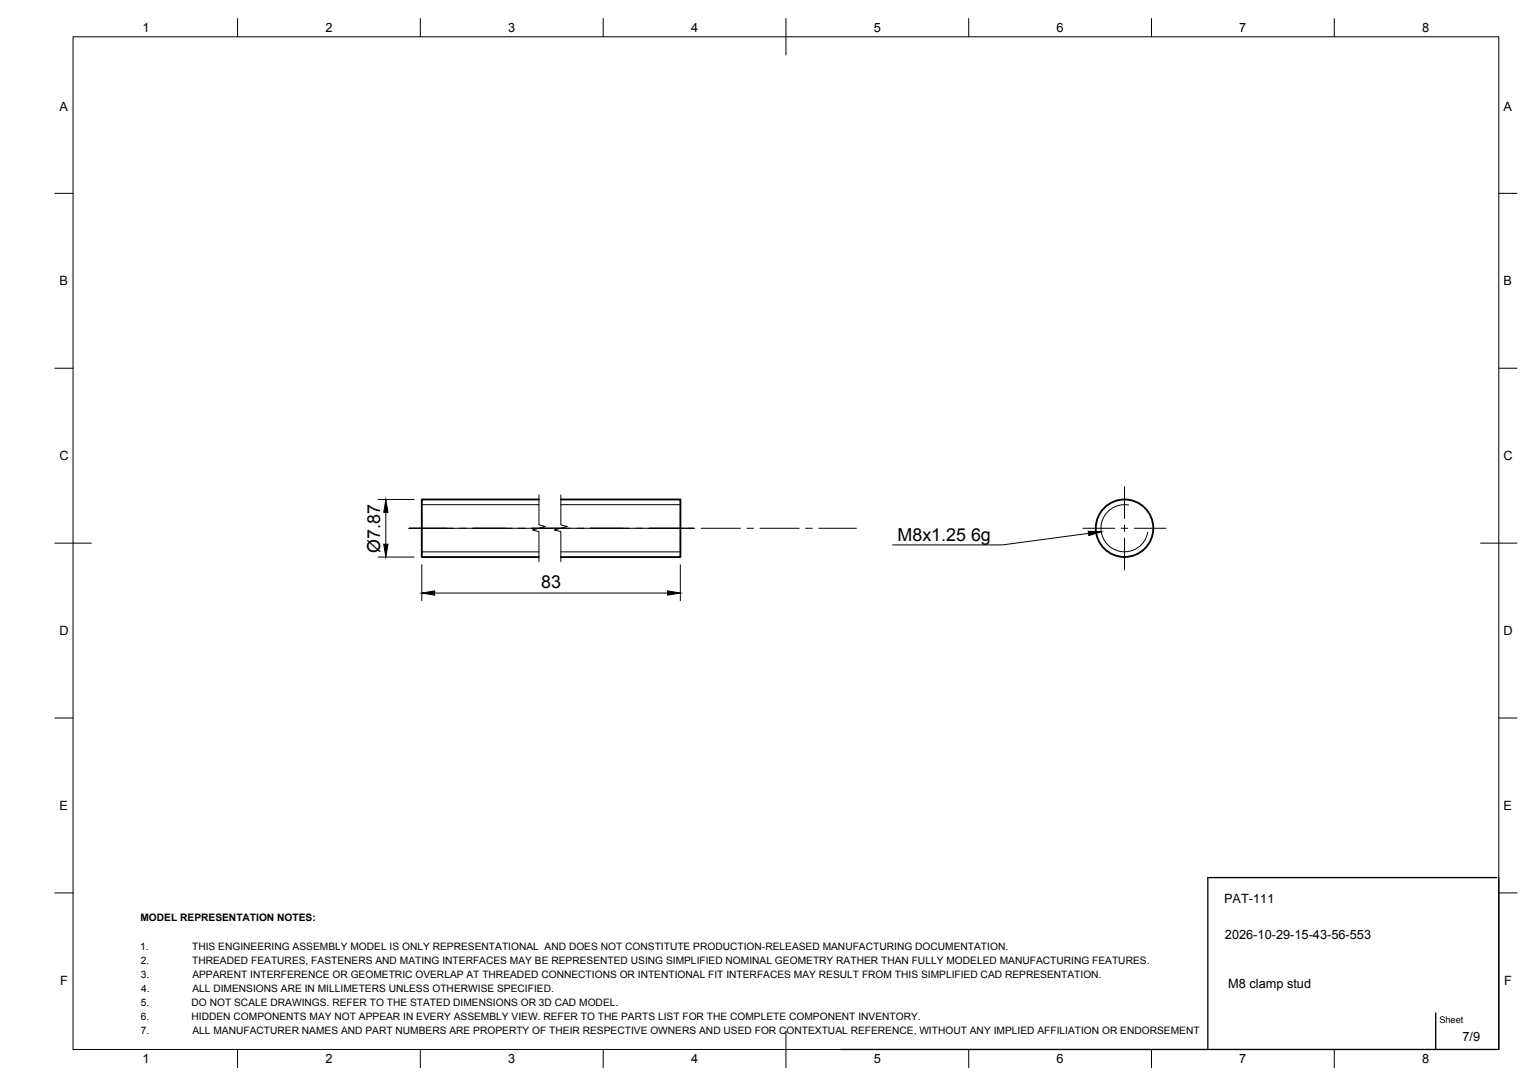
ISO-10303-21;
HEADER;
/* Generated by software containing ST-Developer
 * from STEP Tools, Inc. (www.steptools.com) 
 */

FILE_DESCRIPTION(
/* description */ ('Grid plate located blocks and clamp'),
/* implementation_level */ '2;1');

FILE_NAME(
/* name */ 'M8 clamp stud.step',
/* time_stamp */ '2026-10-29T15:43:47-07:00',
/* author */ (''),
/* organization */ (''),
/* preprocessor_version */ 'ST-DEVELOPER v20.2',
/* originating_system */ 'Autodesk Translation Framework v15.17.0.0',
/* authorisation */ '');

FILE_SCHEMA (('AUTOMOTIVE_DESIGN { 1 0 10303 214 3 1 1 }'));
ENDSEC;

DATA;
#10=MECHANICAL_DESIGN_GEOMETRIC_PRESENTATION_REPRESENTATION('',(#176),#5702);
#150=SHAPE_REPRESENTATION_RELATIONSHIP('SRR','None',#5768,#162);
#162=ADVANCED_BREP_SHAPE_REPRESENTATION('',(#188),#5698);
#176=STYLED_ITEM('',(#5904),#188);
#188=MANIFOLD_SOLID_BREP('Body1',#3273);
#361=CIRCLE('',#3659,0.3933);
#362=CIRCLE('',#3660,0.3933);
#440=CYLINDRICAL_SURFACE('',#3658,0.3933);
#600=FACE_OUTER_BOUND('',#852,.T.);
#601=FACE_OUTER_BOUND('',#853,.T.);
#602=FACE_OUTER_BOUND('',#854,.T.);
#852=EDGE_LOOP('',(#2782,#2783,#2784,#2785));
#853=EDGE_LOOP('',(#2786));
#854=EDGE_LOOP('',(#2787));
#1129=LINE('',#5435,#1402);
#1402=VECTOR('',#4493,0.4);
#1656=VERTEX_POINT('',#5432);
#1657=VERTEX_POINT('',#5434);
#2041=EDGE_CURVE('',#1656,#1656,#361,.F.);
#2042=EDGE_CURVE('',#1656,#1657,#1129,.T.);
#2043=EDGE_CURVE('',#1657,#1657,#362,.F.);
#2782=ORIENTED_EDGE('',*,*,#2041,.F.);
#2783=ORIENTED_EDGE('',*,*,#2042,.T.);
#2784=ORIENTED_EDGE('',*,*,#2043,.T.);
#2785=ORIENTED_EDGE('',*,*,#2042,.F.);
#2786=ORIENTED_EDGE('',*,*,#2041,.T.);
#2787=ORIENTED_EDGE('',*,*,#2043,.F.);
#3057=PLANE('',#3661);
#3058=PLANE('',#3662);
#3221=ADVANCED_FACE('',(#600),#440,.T.);
#3222=ADVANCED_FACE('',(#601),#3057,.T.);
#3223=ADVANCED_FACE('',(#602),#3058,.F.);
#3273=CLOSED_SHELL('',(#3221,#3222,#3223));
#3657=AXIS2_PLACEMENT_3D('',#5430,#4487,#4488);
#3658=AXIS2_PLACEMENT_3D('',#5431,#4489,#4490);
#3659=AXIS2_PLACEMENT_3D('',#5433,#4491,#4492);
#3660=AXIS2_PLACEMENT_3D('',#5436,#4494,#4495);
#3661=AXIS2_PLACEMENT_3D('',#5437,#4496,#4497);
#3662=AXIS2_PLACEMENT_3D('',#5438,#4498,#4499);
#4487=DIRECTION('axis',(0.,0.,1.));
#4488=DIRECTION('refdir',(1.,0.,0.));
#4489=DIRECTION('center_axis',(0.,0.,1.));
#4490=DIRECTION('ref_axis',(1.,0.,0.));
#4491=DIRECTION('center_axis',(0.,0.,-1.));
#4492=DIRECTION('ref_axis',(1.,0.,0.));
#4493=DIRECTION('',(0.,0.,-1.));
#4494=DIRECTION('center_axis',(0.,0.,-1.));
#4495=DIRECTION('ref_axis',(1.,0.,0.));
#4496=DIRECTION('center_axis',(0.,0.,1.));
#4497=DIRECTION('ref_axis',(1.,0.,0.));
#4498=DIRECTION('center_axis',(0.,0.,1.));
#4499=DIRECTION('ref_axis',(1.,0.,0.));
#5430=CARTESIAN_POINT('',(0.,0.,0.));
#5431=CARTESIAN_POINT('Origin',(10.,-4.,0.));
#5432=CARTESIAN_POINT('',(9.6067,-4.,8.3));
#5433=CARTESIAN_POINT('Origin',(10.,-4.,8.3));
#5434=CARTESIAN_POINT('',(9.6067,-4.,0.));
#5435=CARTESIAN_POINT('',(9.6067,-4.,0.));
#5436=CARTESIAN_POINT('Origin',(10.,-4.,0.));
#5437=CARTESIAN_POINT('Origin',(10.,-4.,8.3));
#5438=CARTESIAN_POINT('Origin',(10.,-4.,0.));
#5684=UNCERTAINTY_MEASURE_WITH_UNIT(LENGTH_MEASURE(0.001),#5703,
'DISTANCE_ACCURACY_VALUE',
'Maximum model space distance between geometric entities at asserted c
onnectivities');
#5688=UNCERTAINTY_MEASURE_WITH_UNIT(LENGTH_MEASURE(0.001),#5703,
'DISTANCE_ACCURACY_VALUE',
'Maximum model space distance between geometric entities at asserted c
onnectivities');
#5698=(
GEOMETRIC_REPRESENTATION_CONTEXT(3)
GLOBAL_UNCERTAINTY_ASSIGNED_CONTEXT((#5684))
GLOBAL_UNIT_ASSIGNED_CONTEXT((#5703,#5705,#5706))
REPRESENTATION_CONTEXT('','3D')
);
#5702=(
GEOMETRIC_REPRESENTATION_CONTEXT(3)
GLOBAL_UNCERTAINTY_ASSIGNED_CONTEXT((#5688))
GLOBAL_UNIT_ASSIGNED_CONTEXT((#5703,#5705,#5706))
REPRESENTATION_CONTEXT('','3D')
);
#5703=(
LENGTH_UNIT()
NAMED_UNIT(*)
SI_UNIT(.CENTI.,.METRE.)
);
#5705=(
NAMED_UNIT(*)
PLANE_ANGLE_UNIT()
SI_UNIT($,.RADIAN.)
);
#5706=(
NAMED_UNIT(*)
SI_UNIT($,.STERADIAN.)
SOLID_ANGLE_UNIT()
);
#5716=SHAPE_DEFINITION_REPRESENTATION(#5729,#5768);
#5729=PRODUCT_DEFINITION_SHAPE('',$,#5782);
#5768=SHAPE_REPRESENTATION('',(#3657),#5698);
#5772=PRODUCT_DEFINITION_CONTEXT('part definition',#5813,'design');
#5782=PRODUCT_DEFINITION('M8 clamp stud','M8 clamp stud',#5795,
#5772);
#5795=PRODUCT_DEFINITION_FORMATION('',$,#5824);
#5813=APPLICATION_CONTEXT(
'Core Data for Automotive Mechanical Design Process');
#5814=PRODUCT_CONTEXT('part definition',#5813,'mechanical');
#5824=PRODUCT('M8 clamp stud','M8 clamp stud',
'M8 clamp stud',(#5814));
#5898=COLOUR_RGB('Black',0.12,0.14,0.17);
#5899=FILL_AREA_STYLE_COLOUR('',#5898);
#5900=FILL_AREA_STYLE('',(#5899));
#5901=SURFACE_STYLE_FILL_AREA(#5900);
#5902=SURFACE_SIDE_STYLE('',(#5901));
#5903=SURFACE_STYLE_USAGE(.BOTH.,#5902);
#5904=PRESENTATION_STYLE_ASSIGNMENT((#5903));
ENDSEC;
END-ISO-10303-21;
